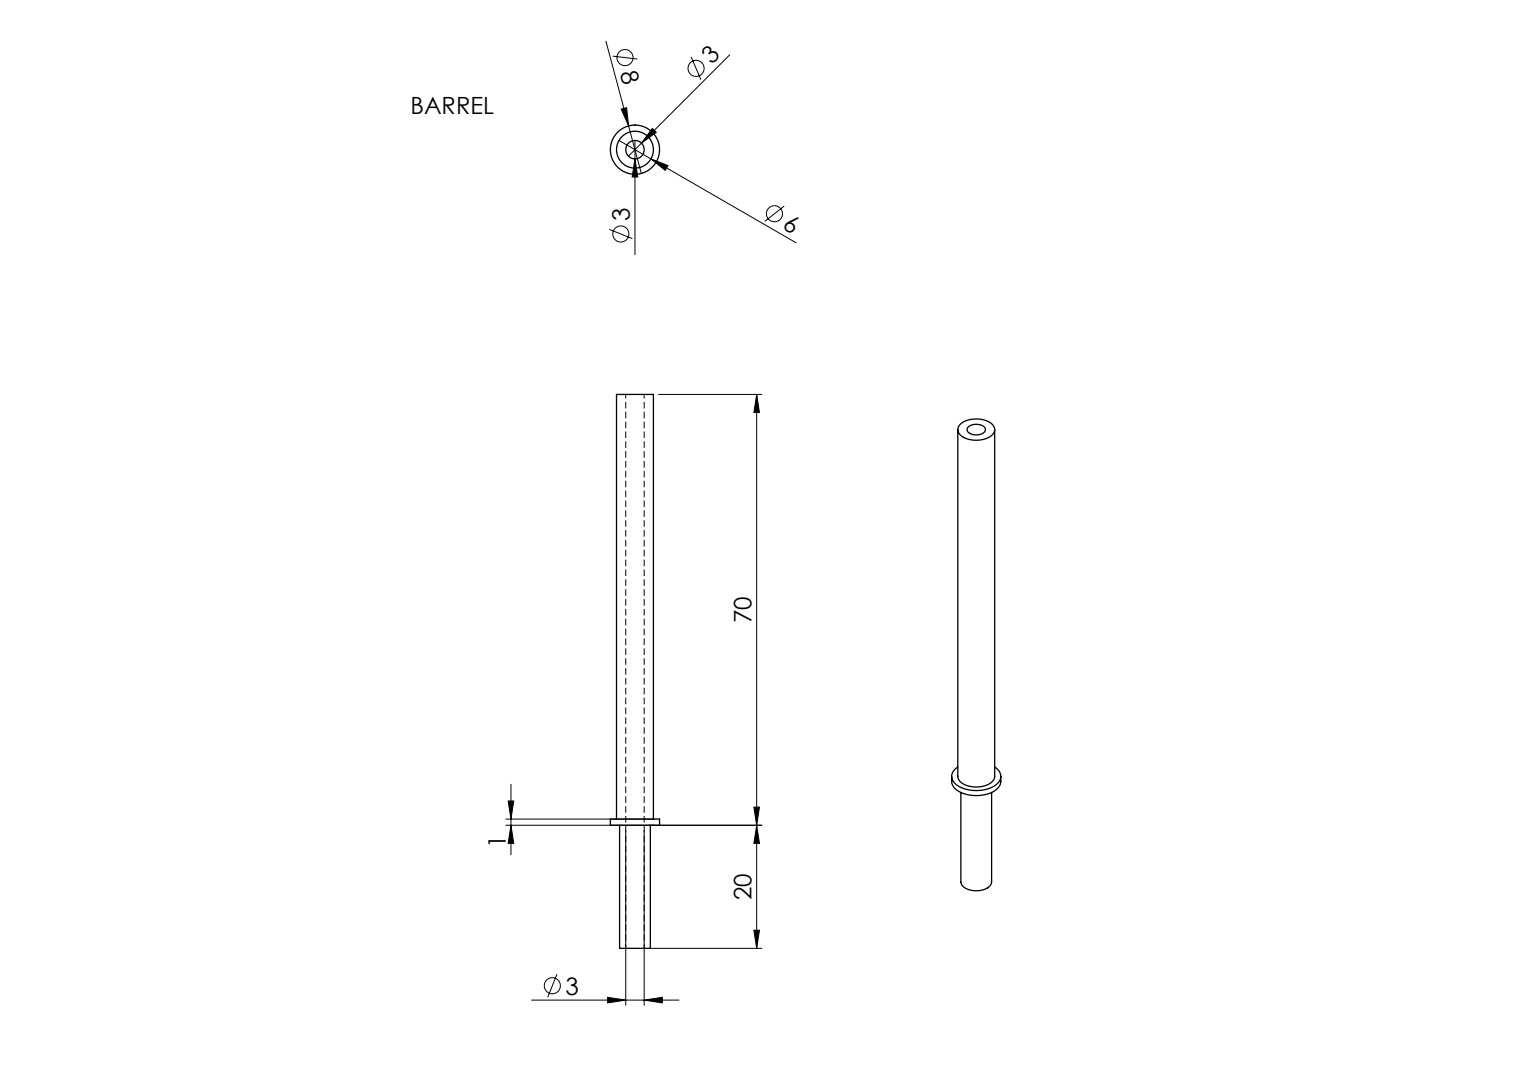
ISO-10303-21;
HEADER;
FILE_DESCRIPTION (('STEP AP214'),
    '1' );
FILE_NAME ('barrel.step',
    '2026-10-27T10:49:47',
    ( '' ),
    ( '' ),
    'SwSTEP 2.0',
    'SolidWorks 2026',
    '' );
FILE_SCHEMA (( 'AUTOMOTIVE_DESIGN' ));
ENDSEC;

DATA;
#22=EDGE_LOOP ( 'NONE', ( #1173, #7087 ) ) ;
#35=ADVANCED_FACE ( 'NONE', ( #4002 ), #1115, .T. ) ;
#54=CIRCLE ( 'NONE', #4368, 3.000000000000000444 ) ;
#95=( NAMED_UNIT ( * ) SI_UNIT ( $, .STERADIAN. ) SOLID_ANGLE_UNIT ( ) );
#116=VERTEX_POINT ( 'NONE', #4866 ) ;
#117=DIRECTION ( 'NONE',  ( 0.000000000000000000, -0.000000000000000000, 1.000000000000000000 ) ) ;
#151=DIRECTION ( 'NONE',  ( 0.000000000000000000, -1.000000000000000000, 0.000000000000000000 ) ) ;
#176=LINE ( 'NONE', #7340, #7480 ) ;
#209=DIRECTION ( 'NONE',  ( 0.000000000000000000, -1.000000000000000000, 0.000000000000000000 ) ) ;
#248=EDGE_CURVE ( 'NONE', #7024, #2834, #3444, .T. ) ;
#261=CARTESIAN_POINT ( 'NONE',  ( 0.000000000000000000, 1.000000000000000000, -3.999999999999999112 ) ) ;
#290=EDGE_CURVE ( 'NONE', #6114, #7024, #5977, .T. ) ;
#326=ORIENTED_EDGE ( 'NONE', *, *, #7017, .T. ) ;
#337=FACE_OUTER_BOUND ( 'NONE', #2501, .T. ) ;
#369=ORIENTED_EDGE ( 'NONE', *, *, #5900, .T. ) ;
#417=ADVANCED_BREP_SHAPE_REPRESENTATION ( '', ( #8468, #888 ), #7729 ) ;
#475=ORIENTED_EDGE ( 'NONE', *, *, #2084, .T. ) ;
#533=CARTESIAN_POINT ( 'NONE',  ( 0.000000000000000000, 70.00000000000000000, 0.000000000000000000 ) ) ;
#572=FACE_OUTER_BOUND ( 'NONE', #9117, .T. ) ;
#618=SURFACE_SIDE_STYLE ('',( #6992 ) ) ;
#623=( NAMED_UNIT ( * ) SI_UNIT ( $, .STERADIAN. ) SOLID_ANGLE_UNIT ( ) );
#637=DIRECTION ( 'NONE',  ( -0.000000000000000000, -1.000000000000000000, -0.000000000000000000 ) ) ;
#651=VECTOR ( 'NONE', #2655, 1000.000000000000000 ) ;
#686=DIRECTION ( 'NONE',  ( 0.000000000000000000, -1.000000000000000000, 0.000000000000000000 ) ) ;
#719=AXIS2_PLACEMENT_3D ( 'NONE', #7347, #8874, #4420 ) ;
#768=EDGE_CURVE ( 'NONE', #2834, #2260, #8516, .T. ) ;
#781=CARTESIAN_POINT ( 'NONE',  ( 3.061616997868383634E-16, -20.00000000000000000, -2.500000000000000444 ) ) ;
#835=ORIENTED_EDGE ( 'NONE', *, *, #8338, .F. ) ;
#878=CARTESIAN_POINT ( 'NONE',  ( 3.673940397442060361E-16, 70.00000000000000000, 3.000000000000000444 ) ) ;
#886=AXIS2_PLACEMENT_3D ( 'NONE', #6121, #3897, #6716 ) ;
#888=AXIS2_PLACEMENT_3D ( 'NONE', #4026, #9081, #6861 ) ;
#899=AXIS2_PLACEMENT_3D ( 'NONE', #5052, #7905, #6359 ) ;
#901=EDGE_CURVE ( 'NONE', #6843, #5960, #176, .T. ) ;
#910=CARTESIAN_POINT ( 'NONE',  ( 0.000000000000000000, 0.000000000000000000, 0.000000000000000000 ) ) ;
#921=CARTESIAN_POINT ( 'NONE',  ( 1.836970198721030181E-16, 70.00000000000000000, 1.500000000000000222 ) ) ;
#973=CARTESIAN_POINT ( 'NONE',  ( 4.898587196589411843E-16, 1.000000000000000000, 3.999999999999999112 ) ) ;
#1002=DIRECTION ( 'NONE',  ( 0.000000000000000000, -1.000000000000000000, 0.000000000000000000 ) ) ;
#1036=DIRECTION ( 'NONE',  ( 0.000000000000000000, 0.000000000000000000, -1.000000000000000000 ) ) ;
#1065=ORIENTED_EDGE ( 'NONE', *, *, #1265, .F. ) ;
#1115=CYLINDRICAL_SURFACE ( 'NONE', #2552, 3.999999999999999112 ) ;
#1139=ORIENTED_EDGE ( 'NONE', *, *, #8338, .T. ) ;
#1173=ORIENTED_EDGE ( 'NONE', *, *, #1265, .T. ) ;
#1220=ORIENTED_EDGE ( 'NONE', *, *, #6666, .T. ) ;
#1235=LINE ( 'NONE', #3240, #2069 ) ;
#1246=ORIENTED_EDGE ( 'NONE', *, *, #6279, .T. ) ;
#1265=EDGE_CURVE ( 'NONE', #2260, #2834, #6581, .T. ) ;
#1271=DIRECTION ( 'NONE',  ( -0.000000000000000000, -1.000000000000000000, -0.000000000000000000 ) ) ;
#1296=CARTESIAN_POINT ( 'NONE',  ( 3.673940397442060361E-16, 1.000000000000000888, 3.000000000000000444 ) ) ;
#1312=DIRECTION ( 'NONE',  ( -0.000000000000000000, -1.000000000000000000, -0.000000000000000000 ) ) ;
#1314=FILL_AREA_STYLE ('',( #8394 ) ) ;
#1334=CIRCLE ( 'NONE', #7748, 1.500000000000000222 ) ;
#1335=EDGE_CURVE ( 'NONE', #8226, #5826, #3482, .T. ) ;
#1339=PRODUCT_DEFINITION_CONTEXT ( 'detailed design', #4961, 'design' ) ;
#1343=AXIS2_PLACEMENT_3D ( 'NONE', #8806, #6806, #1036 ) ;
#1352=CYLINDRICAL_SURFACE ( 'NONE', #1343, 3.999999999999999112 ) ;
#1405=SURFACE_STYLE_USAGE ( .BOTH. , #618 ) ;
#1464=EDGE_CURVE ( 'NONE', #6101, #3013, #5044, .T. ) ;
#1479=CLOSED_SHELL ( 'NONE', ( #4412, #3247, #2822, #5525, #9073, #2667, #4256, #5038, #4493, #35, #5330, #3737 ) ) ;
#1506=EDGE_LOOP ( 'NONE', ( #5687, #3390 ) ) ;
#1527=DIRECTION ( 'NONE',  ( 0.000000000000000000, 1.000000000000000000, 0.000000000000000000 ) ) ;
#1576=ORIENTED_EDGE ( 'NONE', *, *, #1464, .F. ) ;
#1705=FACE_OUTER_BOUND ( 'NONE', #3131, .T. ) ;
#1741=ORIENTED_EDGE ( 'NONE', *, *, #768, .F. ) ;
#1746=CARTESIAN_POINT ( 'NONE',  ( 0.000000000000000000, 70.00000000000000000, 0.000000000000000000 ) ) ;
#1752=VERTEX_POINT ( 'NONE', #7681 ) ;
#1760=CARTESIAN_POINT ( 'NONE',  ( 0.000000000000000000, -20.00000000000000000, 0.000000000000000000 ) ) ;
#1766=CIRCLE ( 'NONE', #719, 2.500000000000000444 ) ;
#1768=ORIENTED_EDGE ( 'NONE', *, *, #2025, .T. ) ;
#1771=CARTESIAN_POINT ( 'NONE',  ( 1.836970198721030181E-16, -20.00000000000000000, 1.500000000000000222 ) ) ;
#1772=EDGE_LOOP ( 'NONE', ( #1220, #9002, #6481, #6040 ) ) ;
#1782=AXIS2_PLACEMENT_3D ( 'NONE', #3671, #1527, #4513 ) ;
#1783=EDGE_LOOP ( 'NONE', ( #3498, #8024, #3217, #7823 ) ) ;
#1815=DIRECTION ( 'NONE',  ( 0.000000000000000000, -1.000000000000000000, 0.000000000000000000 ) ) ;
#1830=EDGE_LOOP ( 'NONE', ( #3630, #6617, #3382, #8852 ) ) ;
#1889=DIRECTION ( 'NONE',  ( 0.000000000000000000, 0.000000000000000000, -1.000000000000000000 ) ) ;
#1906=AXIS2_PLACEMENT_3D ( 'NONE', #2039, #6307, #4863 ) ;
#1909=DIRECTION ( 'NONE',  ( -0.000000000000000000, 1.000000000000000000, -0.000000000000000000 ) ) ;
#1950=CARTESIAN_POINT ( 'NONE',  ( 3.061616997868383634E-16, -20.00000000000000000, -2.500000000000000444 ) ) ;
#1962=CARTESIAN_POINT ( 'NONE',  ( 1.836970198721030181E-16, 70.00000000000000000, 1.500000000000000222 ) ) ;
#1971=LINE ( 'NONE', #4800, #4797 ) ;
#1986=DIRECTION ( 'NONE',  ( 0.000000000000000000, 0.000000000000000000, -1.000000000000000000 ) ) ;
#1990=AXIS2_PLACEMENT_3D ( 'NONE', #8461, #2087, #4227 ) ;
#2025=EDGE_CURVE ( 'NONE', #7863, #6101, #7202, .T. ) ;
#2026=( NAMED_UNIT ( * ) PLANE_ANGLE_UNIT ( ) SI_UNIT ( $, .RADIAN. ) );
#2039=CARTESIAN_POINT ( 'NONE',  ( 0.000000000000000000, 0.000000000000000000, 0.000000000000000000 ) ) ;
#2065=DIRECTION ( 'NONE',  ( 0.000000000000000000, 1.000000000000000000, 0.000000000000000000 ) ) ;
#2069=VECTOR ( 'NONE', #7469, 1000.000000000000000 ) ;
#2083=VECTOR ( 'NONE', #6598, 1000.000000000000000 ) ;
#2084=EDGE_CURVE ( 'NONE', #5960, #5957, #3878, .T. ) ;
#2087=DIRECTION ( 'NONE',  ( 0.000000000000000000, -1.000000000000000000, 0.000000000000000000 ) ) ;
#2156=CYLINDRICAL_SURFACE ( 'NONE', #4658, 1.500000000000000222 ) ;
#2260=VERTEX_POINT ( 'NONE', #8456 ) ;
#2273=DIRECTION ( 'NONE',  ( -0.000000000000000000, -1.000000000000000000, -0.000000000000000000 ) ) ;
#2276=ORIENTED_EDGE ( 'NONE', *, *, #7313, .F. ) ;
#2297=EDGE_CURVE ( 'NONE', #7186, #8226, #1334, .T. ) ;
#2310=DIRECTION ( 'NONE',  ( 0.000000000000000000, 1.000000000000000000, 0.000000000000000000 ) ) ;
#2334=CARTESIAN_POINT ( 'NONE',  ( 0.000000000000000000, -20.00000000000000000, -1.500000000000000222 ) ) ;
#2347=ORIENTED_EDGE ( 'NONE', *, *, #2994, .T. ) ;
#2360=CIRCLE ( 'NONE', #3409, 1.500000000000000222 ) ;
#2381=AXIS2_PLACEMENT_3D ( 'NONE', #8404, #6381, #1986 ) ;
#2460=DIRECTION ( 'NONE',  ( 1.000000000000000000, 0.000000000000000000, 0.000000000000000000 ) ) ;
#2501=EDGE_LOOP ( 'NONE', ( #7351, #2982, #1065, #4344 ) ) ;
#2541=DIRECTION ( 'NONE',  ( 0.000000000000000000, 0.000000000000000000, 1.000000000000000000 ) ) ;
#2552=AXIS2_PLACEMENT_3D ( 'NONE', #6080, #1815, #3168 ) ;
#2585=FACE_BOUND ( 'NONE', #4396, .T. ) ;
#2612=CARTESIAN_POINT ( 'NONE',  ( 0.000000000000000000, -20.00000000000000000, 0.000000000000000000 ) ) ;
#2616=SHAPE_DEFINITION_REPRESENTATION ( #4672, #3200 ) ;
#2655=DIRECTION ( 'NONE',  ( 0.000000000000000000, -1.000000000000000000, 0.000000000000000000 ) ) ;
#2667=ADVANCED_FACE ( 'NONE', ( #1705, #6583 ), #7375, .T. ) ;
#2697=VECTOR ( 'NONE', #4369, 1000.000000000000000 ) ;
#2741=AXIS2_PLACEMENT_3D ( 'NONE', #6157, #3930, #4669 ) ;
#2788=CARTESIAN_POINT ( 'NONE',  ( 0.000000000000000000, 70.00000000000000000, 0.000000000000000000 ) ) ;
#2822=ADVANCED_FACE ( 'NONE', ( #3293 ), #4681, .F. ) ;
#2834=VERTEX_POINT ( 'NONE', #5371 ) ;
#2864=FACE_OUTER_BOUND ( 'NONE', #22, .T. ) ;
#2928=CARTESIAN_POINT ( 'NONE',  ( 3.061616997868383634E-16, 0.000000000000000000, -2.500000000000000444 ) ) ;
#2945=PRODUCT_DEFINITION_FORMATION_WITH_SPECIFIED_SOURCE ( 'ANY', '', #8393, .NOT_KNOWN. ) ;
#2948=MECHANICAL_DESIGN_GEOMETRIC_PRESENTATION_REPRESENTATION('',(#5632),#3563);
#2959=ORIENTED_EDGE ( 'NONE', *, *, #7430, .T. ) ;
#2960=ORIENTED_EDGE ( 'NONE', *, *, #6666, .F. ) ;
#2982=ORIENTED_EDGE ( 'NONE', *, *, #248, .T. ) ;
#2994=EDGE_CURVE ( 'NONE', #7024, #6114, #3567, .T. ) ;
#3001=DIRECTION ( 'NONE',  ( 0.000000000000000000, -0.000000000000000000, -1.000000000000000000 ) ) ;
#3013=VERTEX_POINT ( 'NONE', #4897 ) ;
#3051=DIRECTION ( 'NONE',  ( -0.000000000000000000, 1.000000000000000000, -0.000000000000000000 ) ) ;
#3092=FACE_OUTER_BOUND ( 'NONE', #1506, .T. ) ;
#3095=CARTESIAN_POINT ( 'NONE',  ( 0.000000000000000000, 1.000000000000000888, 0.000000000000000000 ) ) ;
#3131=EDGE_LOOP ( 'NONE', ( #8535, #369 ) ) ;
#3168=DIRECTION ( 'NONE',  ( 0.000000000000000000, 0.000000000000000000, -1.000000000000000000 ) ) ;
#3180=CIRCLE ( 'NONE', #4212, 3.000000000000000444 ) ;
#3191=DIRECTION ( 'NONE',  ( 0.000000000000000000, -1.000000000000000000, 0.000000000000000000 ) ) ;
#3200=SHAPE_REPRESENTATION ( 'barrel', ( #888 ), #7729 ) ;
#3217=ORIENTED_EDGE ( 'NONE', *, *, #5142, .F. ) ;
#3240=CARTESIAN_POINT ( 'NONE',  ( 0.000000000000000000, -20.00000000000000000, 2.500000000000000444 ) ) ;
#3247=ADVANCED_FACE ( 'NONE', ( #337 ), #1352, .T. ) ;
#3258=CARTESIAN_POINT ( 'NONE',  ( 0.000000000000000000, 70.00000000000000000, 0.000000000000000000 ) ) ;
#3263=ORIENTED_EDGE ( 'NONE', *, *, #248, .F. ) ;
#3274=AXIS2_PLACEMENT_3D ( 'NONE', #5839, #2310, #117 ) ;
#3278=EDGE_CURVE ( 'NONE', #5826, #6937, #5346, .T. ) ;
#3279=COLOUR_RGB ( '',0.8941176470588234615, 0.8941176470588234615, 0.8941176470588234615 ) ;
#3293=FACE_OUTER_BOUND ( 'NONE', #1772, .T. ) ;
#3302=FACE_OUTER_BOUND ( 'NONE', #6606, .T. ) ;
#3382=ORIENTED_EDGE ( 'NONE', *, *, #4776, .T. ) ;
#3390=ORIENTED_EDGE ( 'NONE', *, *, #2994, .F. ) ;
#3409=AXIS2_PLACEMENT_3D ( 'NONE', #1746, #6762, #2541 ) ;
#3420=( NAMED_UNIT ( * ) PLANE_ANGLE_UNIT ( ) SI_UNIT ( $, .RADIAN. ) );
#3444=LINE ( 'NONE', #5613, #8804 ) ;
#3460=DIRECTION ( 'NONE',  ( 0.000000000000000000, 0.000000000000000000, -1.000000000000000000 ) ) ;
#3466=PLANE ( 'NONE',  #3609 ) ;
#3482=LINE ( 'NONE', #3615, #4273 ) ;
#3486=PRODUCT_DEFINITION ( 'UNKNOWN', '', #2945, #1339 ) ;
#3498=ORIENTED_EDGE ( 'NONE', *, *, #5900, .F. ) ;
#3510=( LENGTH_UNIT ( ) NAMED_UNIT ( * ) SI_UNIT ( .MILLI., .METRE. ) );
#3547=CIRCLE ( 'NONE', #7110, 1.500000000000000222 ) ;
#3563=( GEOMETRIC_REPRESENTATION_CONTEXT ( 3 ) GLOBAL_UNCERTAINTY_ASSIGNED_CONTEXT ( ( #7291 ) ) GLOBAL_UNIT_ASSIGNED_CONTEXT ( ( #3510, #2026, #623 ) ) REPRESENTATION_CONTEXT ( 'NONE', 'WORKASPACE' ) );
#3567=CIRCLE ( 'NONE', #2381, 3.999999999999999112 ) ;
#3609=AXIS2_PLACEMENT_3D ( 'NONE', #9087, #2065, #5021 ) ;
#3615=CARTESIAN_POINT ( 'NONE',  ( 0.000000000000000000, 70.00000000000000000, -1.500000000000000222 ) ) ;
#3630=ORIENTED_EDGE ( 'NONE', *, *, #901, .F. ) ;
#3671=CARTESIAN_POINT ( 'NONE',  ( 0.000000000000000000, 70.00000000000000000, 0.000000000000000000 ) ) ;
#3675=MECHANICAL_DESIGN_GEOMETRIC_PRESENTATION_REPRESENTATION('',(#9162),#7384);
#3737=ADVANCED_FACE ( 'NONE', ( #3302 ), #8963, .T. ) ;
#3751=DIRECTION ( 'NONE',  ( 1.000000000000000000, 0.000000000000000000, 0.000000000000000000 ) ) ;
#3775=AXIS2_PLACEMENT_3D ( 'NONE', #8021, #209, #3751 ) ;
#3806=EDGE_LOOP ( 'NONE', ( #2960, #7095 ) ) ;
#3878=CIRCLE ( 'NONE', #899, 3.000000000000000444 ) ;
#3897=DIRECTION ( 'NONE',  ( -0.000000000000000000, -1.000000000000000000, -0.000000000000000000 ) ) ;
#3930=DIRECTION ( 'NONE',  ( 0.000000000000000000, -1.000000000000000000, 0.000000000000000000 ) ) ;
#3931=CIRCLE ( 'NONE', #3775, 2.500000000000000444 ) ;
#3989=ORIENTED_EDGE ( 'NONE', *, *, #9010, .F. ) ;
#4001=LINE ( 'NONE', #8138, #651 ) ;
#4002=FACE_OUTER_BOUND ( 'NONE', #4221, .T. ) ;
#4026=CARTESIAN_POINT ( 'NONE',  ( 0.000000000000000000, 0.000000000000000000, 0.000000000000000000 ) ) ;
#4056=ORIENTED_EDGE ( 'NONE', *, *, #2297, .T. ) ;
#4157=CYLINDRICAL_SURFACE ( 'NONE', #6087, 3.000000000000000444 ) ;
#4164=FACE_OUTER_BOUND ( 'NONE', #5923, .T. ) ;
#4198=CARTESIAN_POINT ( 'NONE',  ( 0.000000000000000000, 70.00000000000000000, 0.000000000000000000 ) ) ;
#4212=AXIS2_PLACEMENT_3D ( 'NONE', #3095, #8665, #6010 ) ;
#4221=EDGE_LOOP ( 'NONE', ( #3263, #2347, #5735, #1741 ) ) ;
#4227=DIRECTION ( 'NONE',  ( 0.000000000000000000, 0.000000000000000000, -1.000000000000000000 ) ) ;
#4256=ADVANCED_FACE ( 'NONE', ( #6376, #2864 ), #3466, .F. ) ;
#4273=VECTOR ( 'NONE', #637, 1000.000000000000000 ) ;
#4318=CARTESIAN_POINT ( 'NONE',  ( 0.000000000000000000, -20.00000000000000000, 0.000000000000000000 ) ) ;
#4334=CYLINDRICAL_SURFACE ( 'NONE', #4517, 3.000000000000000444 ) ;
#4344=ORIENTED_EDGE ( 'NONE', *, *, #5766, .F. ) ;
#4368=AXIS2_PLACEMENT_3D ( 'NONE', #3258, #6083, #8919 ) ;
#4369=DIRECTION ( 'NONE',  ( -0.000000000000000000, 1.000000000000000000, -0.000000000000000000 ) ) ;
#4382=PRESENTATION_STYLE_ASSIGNMENT (( #1405 ) ) ;
#4396=EDGE_LOOP ( 'NONE', ( #6921, #2276 ) ) ;
#4412=ADVANCED_FACE ( 'NONE', ( #4164 ), #6998, .T. ) ;
#4420=DIRECTION ( 'NONE',  ( 1.000000000000000000, 0.000000000000000000, 0.000000000000000000 ) ) ;
#4493=ADVANCED_FACE ( 'NONE', ( #3092, #7176 ), #5772, .F. ) ;
#4513=DIRECTION ( 'NONE',  ( 0.000000000000000000, 0.000000000000000000, 1.000000000000000000 ) ) ;
#4517=AXIS2_PLACEMENT_3D ( 'NONE', #4198, #1312, #7166 ) ;
#4658=AXIS2_PLACEMENT_3D ( 'NONE', #8527, #4934, #6293 ) ;
#4669=DIRECTION ( 'NONE',  ( 0.000000000000000000, -0.000000000000000000, -1.000000000000000000 ) ) ;
#4672=PRODUCT_DEFINITION_SHAPE ( 'NONE', 'NONE',  #3486 ) ;
#4681=CYLINDRICAL_SURFACE ( 'NONE', #886, 1.500000000000000222 ) ;
#4700=ORIENTED_EDGE ( 'NONE', *, *, #2025, .F. ) ;
#4734=DIRECTION ( 'NONE',  ( 0.000000000000000000, 0.000000000000000000, 1.000000000000000000 ) ) ;
#4776=EDGE_CURVE ( 'NONE', #1752, #5957, #1971, .T. ) ;
#4785=PRODUCT_CONTEXT ( 'NONE', #5448, 'mechanical' ) ;
#4797=VECTOR ( 'NONE', #1271, 1000.000000000000000 ) ;
#4800=CARTESIAN_POINT ( 'NONE',  ( 0.000000000000000000, 70.00000000000000000, -3.000000000000000444 ) ) ;
#4863=DIRECTION ( 'NONE',  ( 0.000000000000000000, 0.000000000000000000, -1.000000000000000000 ) ) ;
#4866=CARTESIAN_POINT ( 'NONE',  ( 0.000000000000000000, -20.00000000000000000, 2.500000000000000444 ) ) ;
#4878=CARTESIAN_POINT ( 'NONE',  ( 0.000000000000000000, -20.00000000000000000, 0.000000000000000000 ) ) ;
#4897=CARTESIAN_POINT ( 'NONE',  ( 0.000000000000000000, 0.000000000000000000, 2.500000000000000444 ) ) ;
#4934=DIRECTION ( 'NONE',  ( -0.000000000000000000, -1.000000000000000000, -0.000000000000000000 ) ) ;
#4961=APPLICATION_CONTEXT ( 'automotive_design' ) ;
#5021=DIRECTION ( 'NONE',  ( 0.000000000000000000, -0.000000000000000000, 1.000000000000000000 ) ) ;
#5038=ADVANCED_FACE ( 'NONE', ( #7040 ), #2156, .F. ) ;
#5044=CIRCLE ( 'NONE', #8916, 2.500000000000000444 ) ;
#5052=CARTESIAN_POINT ( 'NONE',  ( 0.000000000000000000, 1.000000000000000888, 0.000000000000000000 ) ) ;
#5060=ORIENTED_EDGE ( 'NONE', *, *, #6279, .F. ) ;
#5084=AXIS2_PLACEMENT_3D ( 'NONE', #5639, #3051, #5868 ) ;
#5142=EDGE_CURVE ( 'NONE', #5957, #5960, #3180, .T. ) ;
#5287=DIRECTION ( 'NONE',  ( 0.000000000000000000, 0.000000000000000000, -1.000000000000000000 ) ) ;
#5330=ADVANCED_FACE ( 'NONE', ( #572, #2585 ), #9031, .T. ) ;
#5346=CIRCLE ( 'NONE', #6093, 1.500000000000000222 ) ;
#5371=CARTESIAN_POINT ( 'NONE',  ( 4.898587196589411843E-16, 0.000000000000000000, 3.999999999999999112 ) ) ;
#5448=APPLICATION_CONTEXT ( 'automotive_design' ) ;
#5507=FACE_OUTER_BOUND ( 'NONE', #1830, .T. ) ;
#5525=ADVANCED_FACE ( 'NONE', ( #8562 ), #4334, .T. ) ;
#5530=DIRECTION ( 'NONE',  ( 0.000000000000000000, -1.000000000000000000, 0.000000000000000000 ) ) ;
#5613=CARTESIAN_POINT ( 'NONE',  ( 4.898587196589411843E-16, 1.000000000000000000, 3.999999999999999112 ) ) ;
#5632=STYLED_ITEM('',(#9218),#8468);
#5633=SHAPE_REPRESENTATION_RELATIONSHIP ( 'NONE' , 'NONE' ,  #3200, #417 ) ;
#5639=CARTESIAN_POINT ( 'NONE',  ( 0.000000000000000000, -20.00000000000000000, 0.000000000000000000 ) ) ;
#5687=ORIENTED_EDGE ( 'NONE', *, *, #290, .F. ) ;
#5735=ORIENTED_EDGE ( 'NONE', *, *, #5766, .T. ) ;
#5766=EDGE_CURVE ( 'NONE', #6114, #2260, #4001, .T. ) ;
#5772=PLANE ( 'NONE',  #6282 ) ;
#5818=( LENGTH_UNIT ( ) NAMED_UNIT ( * ) SI_UNIT ( .MILLI., .METRE. ) );
#5826=VERTEX_POINT ( 'NONE', #2334 ) ;
#5837=CARTESIAN_POINT ( 'NONE',  ( 0.000000000000000000, 70.00000000000000000, -1.500000000000000222 ) ) ;
#5839=CARTESIAN_POINT ( 'NONE',  ( 0.000000000000000000, 70.00000000000000000, 0.000000000000000000 ) ) ;
#5868=DIRECTION ( 'NONE',  ( 0.000000000000000000, 0.000000000000000000, 1.000000000000000000 ) ) ;
#5891=UNCERTAINTY_MEASURE_WITH_UNIT (LENGTH_MEASURE( 1.000000000000000082E-05 ), #6946, 'distance_accuracy_value', 'NONE');
#5900=EDGE_CURVE ( 'NONE', #6843, #1752, #54, .T. ) ;
#5923=EDGE_LOOP ( 'NONE', ( #9154, #1768, #7664, #835 ) ) ;
#5957=VERTEX_POINT ( 'NONE', #7060 ) ;
#5960=VERTEX_POINT ( 'NONE', #1296 ) ;
#5975=DIRECTION ( 'NONE',  ( 1.000000000000000000, 0.000000000000000000, 0.000000000000000000 ) ) ;
#5977=CIRCLE ( 'NONE', #1990, 3.999999999999999112 ) ;
#6010=DIRECTION ( 'NONE',  ( 0.000000000000000000, 0.000000000000000000, -1.000000000000000000 ) ) ;
#6040=ORIENTED_EDGE ( 'NONE', *, *, #1335, .F. ) ;
#6080=CARTESIAN_POINT ( 'NONE',  ( 0.000000000000000000, 1.000000000000000000, 0.000000000000000000 ) ) ;
#6083=DIRECTION ( 'NONE',  ( 0.000000000000000000, 1.000000000000000000, 0.000000000000000000 ) ) ;
#6087=AXIS2_PLACEMENT_3D ( 'NONE', #533, #6161, #3460 ) ;
#6093=AXIS2_PLACEMENT_3D ( 'NONE', #4878, #3191, #1889 ) ;
#6101=VERTEX_POINT ( 'NONE', #2928 ) ;
#6114=VERTEX_POINT ( 'NONE', #261 ) ;
#6121=CARTESIAN_POINT ( 'NONE',  ( 0.000000000000000000, 70.00000000000000000, 0.000000000000000000 ) ) ;
#6157=CARTESIAN_POINT ( 'NONE',  ( 0.000000000000000000, -20.00000000000000000, 0.000000000000000000 ) ) ;
#6161=DIRECTION ( 'NONE',  ( -0.000000000000000000, -1.000000000000000000, -0.000000000000000000 ) ) ;
#6279=EDGE_CURVE ( 'NONE', #116, #7863, #3931, .T. ) ;
#6282=AXIS2_PLACEMENT_3D ( 'NONE', #6514, #151, #3001 ) ;
#6293=DIRECTION ( 'NONE',  ( 0.000000000000000000, 0.000000000000000000, -1.000000000000000000 ) ) ;
#6307=DIRECTION ( 'NONE',  ( 0.000000000000000000, -1.000000000000000000, 0.000000000000000000 ) ) ;
#6314=DIRECTION ( 'NONE',  ( 0.000000000000000000, 0.000000000000000000, -1.000000000000000000 ) ) ;
#6359=DIRECTION ( 'NONE',  ( 0.000000000000000000, 0.000000000000000000, -1.000000000000000000 ) ) ;
#6376=FACE_BOUND ( 'NONE', #7465, .T. ) ;
#6381=DIRECTION ( 'NONE',  ( 0.000000000000000000, -1.000000000000000000, 0.000000000000000000 ) ) ;
#6436=ORIENTED_EDGE ( 'NONE', *, *, #1335, .T. ) ;
#6481=ORIENTED_EDGE ( 'NONE', *, *, #7313, .T. ) ;
#6514=CARTESIAN_POINT ( 'NONE',  ( 0.000000000000000000, 1.000000000000000000, 0.000000000000000000 ) ) ;
#6539=UNCERTAINTY_MEASURE_WITH_UNIT (LENGTH_MEASURE( 1.000000000000000082E-05 ), #5818, 'distance_accuracy_value', 'NONE');
#6581=CIRCLE ( 'NONE', #1906, 3.999999999999999112 ) ;
#6583=FACE_BOUND ( 'NONE', #3806, .T. ) ;
#6598=DIRECTION ( 'NONE',  ( -0.000000000000000000, -1.000000000000000000, -0.000000000000000000 ) ) ;
#6606=EDGE_LOOP ( 'NONE', ( #4700, #5060, #1139, #326 ) ) ;
#6617=ORIENTED_EDGE ( 'NONE', *, *, #8913, .F. ) ;
#6637=DIRECTION ( 'NONE',  ( 0.000000000000000000, -1.000000000000000000, 0.000000000000000000 ) ) ;
#6663=AXIS2_PLACEMENT_3D ( 'NONE', #1760, #7434, #2460 ) ;
#6664=EDGE_LOOP ( 'NONE', ( #8316, #475 ) ) ;
#6666=EDGE_CURVE ( 'NONE', #8226, #7186, #2360, .T. ) ;
#6716=DIRECTION ( 'NONE',  ( 0.000000000000000000, 0.000000000000000000, -1.000000000000000000 ) ) ;
#6762=DIRECTION ( 'NONE',  ( 0.000000000000000000, 1.000000000000000000, 0.000000000000000000 ) ) ;
#6806=DIRECTION ( 'NONE',  ( 0.000000000000000000, -1.000000000000000000, 0.000000000000000000 ) ) ;
#6843=VERTEX_POINT ( 'NONE', #878 ) ;
#6861=DIRECTION ( 'NONE',  ( 1.000000000000000000, 0.000000000000000000, 0.000000000000000000 ) ) ;
#6901=ORIENTED_EDGE ( 'NONE', *, *, #7017, .F. ) ;
#6921=ORIENTED_EDGE ( 'NONE', *, *, #3278, .F. ) ;
#6937=VERTEX_POINT ( 'NONE', #1771 ) ;
#6946=( LENGTH_UNIT ( ) NAMED_UNIT ( * ) SI_UNIT ( .MILLI., .METRE. ) );
#6992=SURFACE_STYLE_FILL_AREA ( #1314 ) ;
#6998=CYLINDRICAL_SURFACE ( 'NONE', #5084, 2.500000000000000444 ) ;
#7017=EDGE_CURVE ( 'NONE', #3013, #6101, #1766, .T. ) ;
#7024=VERTEX_POINT ( 'NONE', #973 ) ;
#7040=FACE_OUTER_BOUND ( 'NONE', #8700, .T. ) ;
#7054=DIRECTION ( 'NONE',  ( 0.000000000000000000, 1.000000000000000000, 0.000000000000000000 ) ) ;
#7060=CARTESIAN_POINT ( 'NONE',  ( 0.000000000000000000, 1.000000000000000888, -3.000000000000000444 ) ) ;
#7087=ORIENTED_EDGE ( 'NONE', *, *, #768, .T. ) ;
#7095=ORIENTED_EDGE ( 'NONE', *, *, #2297, .F. ) ;
#7110=AXIS2_PLACEMENT_3D ( 'NONE', #4318, #686, #6314 ) ;
#7166=DIRECTION ( 'NONE',  ( 0.000000000000000000, 0.000000000000000000, -1.000000000000000000 ) ) ;
#7170=( NAMED_UNIT ( * ) PLANE_ANGLE_UNIT ( ) SI_UNIT ( $, .RADIAN. ) );
#7175=AXIS2_PLACEMENT_3D ( 'NONE', #8039, #6637, #5287 ) ;
#7176=FACE_BOUND ( 'NONE', #6664, .T. ) ;
#7186=VERTEX_POINT ( 'NONE', #1962 ) ;
#7202=LINE ( 'NONE', #781, #2697 ) ;
#7291=UNCERTAINTY_MEASURE_WITH_UNIT (LENGTH_MEASURE( 1.000000000000000082E-05 ), #3510, 'distance_accuracy_value', 'NONE');
#7297=LINE ( 'NONE', #921, #2083 ) ;
#7313=EDGE_CURVE ( 'NONE', #6937, #5826, #3547, .T. ) ;
#7340=CARTESIAN_POINT ( 'NONE',  ( 3.673940397442060361E-16, 70.00000000000000000, 3.000000000000000444 ) ) ;
#7347=CARTESIAN_POINT ( 'NONE',  ( 0.000000000000000000, 0.000000000000000000, 0.000000000000000000 ) ) ;
#7351=ORIENTED_EDGE ( 'NONE', *, *, #290, .T. ) ;
#7375=PLANE ( 'NONE',  #3274 ) ;
#7384=( GEOMETRIC_REPRESENTATION_CONTEXT ( 3 ) GLOBAL_UNCERTAINTY_ASSIGNED_CONTEXT ( ( #6539 ) ) GLOBAL_UNIT_ASSIGNED_CONTEXT ( ( #5818, #7170, #95 ) ) REPRESENTATION_CONTEXT ( 'NONE', 'WORKASPACE' ) );
#7430=EDGE_CURVE ( 'NONE', #7863, #116, #8004, .T. ) ;
#7434=DIRECTION ( 'NONE',  ( 0.000000000000000000, -1.000000000000000000, 0.000000000000000000 ) ) ;
#7465=EDGE_LOOP ( 'NONE', ( #6901, #1576 ) ) ;
#7469=DIRECTION ( 'NONE',  ( -0.000000000000000000, 1.000000000000000000, -0.000000000000000000 ) ) ;
#7480=VECTOR ( 'NONE', #2273, 1000.000000000000000 ) ;
#7556=( NAMED_UNIT ( * ) SI_UNIT ( $, .STERADIAN. ) SOLID_ANGLE_UNIT ( ) );
#7664=ORIENTED_EDGE ( 'NONE', *, *, #1464, .T. ) ;
#7681=CARTESIAN_POINT ( 'NONE',  ( 0.000000000000000000, 70.00000000000000000, -3.000000000000000444 ) ) ;
#7729=( GEOMETRIC_REPRESENTATION_CONTEXT ( 3 ) GLOBAL_UNCERTAINTY_ASSIGNED_CONTEXT ( ( #5891 ) ) GLOBAL_UNIT_ASSIGNED_CONTEXT ( ( #6946, #3420, #7556 ) ) REPRESENTATION_CONTEXT ( 'NONE', 'WORKASPACE' ) );
#7748=AXIS2_PLACEMENT_3D ( 'NONE', #2788, #7054, #8502 ) ;
#7823=ORIENTED_EDGE ( 'NONE', *, *, #4776, .F. ) ;
#7863=VERTEX_POINT ( 'NONE', #1950 ) ;
#7905=DIRECTION ( 'NONE',  ( 0.000000000000000000, -1.000000000000000000, 0.000000000000000000 ) ) ;
#8004=CIRCLE ( 'NONE', #6663, 2.500000000000000444 ) ;
#8021=CARTESIAN_POINT ( 'NONE',  ( 0.000000000000000000, -20.00000000000000000, 0.000000000000000000 ) ) ;
#8024=ORIENTED_EDGE ( 'NONE', *, *, #901, .T. ) ;
#8039=CARTESIAN_POINT ( 'NONE',  ( 0.000000000000000000, 0.000000000000000000, 0.000000000000000000 ) ) ;
#8138=CARTESIAN_POINT ( 'NONE',  ( 0.000000000000000000, 1.000000000000000000, -3.999999999999999112 ) ) ;
#8226=VERTEX_POINT ( 'NONE', #5837 ) ;
#8316=ORIENTED_EDGE ( 'NONE', *, *, #5142, .T. ) ;
#8327=AXIS2_PLACEMENT_3D ( 'NONE', #2612, #1909, #4734 ) ;
#8338=EDGE_CURVE ( 'NONE', #116, #3013, #1235, .T. ) ;
#8393=PRODUCT ( 'barrel', 'barrel', '', ( #4785 ) ) ;
#8394=FILL_AREA_STYLE_COLOUR ( '', #3279 ) ;
#8404=CARTESIAN_POINT ( 'NONE',  ( 0.000000000000000000, 1.000000000000000000, 0.000000000000000000 ) ) ;
#8456=CARTESIAN_POINT ( 'NONE',  ( 0.000000000000000000, 0.000000000000000000, -3.999999999999999112 ) ) ;
#8461=CARTESIAN_POINT ( 'NONE',  ( 0.000000000000000000, 1.000000000000000000, 0.000000000000000000 ) ) ;
#8468=MANIFOLD_SOLID_BREP ( 'Extrude-Thin1', #1479 ) ;
#8502=DIRECTION ( 'NONE',  ( 0.000000000000000000, 0.000000000000000000, 1.000000000000000000 ) ) ;
#8516=CIRCLE ( 'NONE', #7175, 3.999999999999999112 ) ;
#8527=CARTESIAN_POINT ( 'NONE',  ( 0.000000000000000000, 70.00000000000000000, 0.000000000000000000 ) ) ;
#8535=ORIENTED_EDGE ( 'NONE', *, *, #8913, .T. ) ;
#8562=FACE_OUTER_BOUND ( 'NONE', #1783, .T. ) ;
#8609=CIRCLE ( 'NONE', #1782, 3.000000000000000444 ) ;
#8665=DIRECTION ( 'NONE',  ( 0.000000000000000000, -1.000000000000000000, 0.000000000000000000 ) ) ;
#8697=ORIENTED_EDGE ( 'NONE', *, *, #3278, .T. ) ;
#8700=EDGE_LOOP ( 'NONE', ( #3989, #4056, #6436, #8697 ) ) ;
#8804=VECTOR ( 'NONE', #5530, 1000.000000000000000 ) ;
#8806=CARTESIAN_POINT ( 'NONE',  ( 0.000000000000000000, 1.000000000000000000, 0.000000000000000000 ) ) ;
#8852=ORIENTED_EDGE ( 'NONE', *, *, #2084, .F. ) ;
#8874=DIRECTION ( 'NONE',  ( 0.000000000000000000, -1.000000000000000000, 0.000000000000000000 ) ) ;
#8913=EDGE_CURVE ( 'NONE', #1752, #6843, #8609, .T. ) ;
#8916=AXIS2_PLACEMENT_3D ( 'NONE', #910, #1002, #5975 ) ;
#8919=DIRECTION ( 'NONE',  ( 0.000000000000000000, 0.000000000000000000, 1.000000000000000000 ) ) ;
#8963=CYLINDRICAL_SURFACE ( 'NONE', #8327, 2.500000000000000444 ) ;
#9002=ORIENTED_EDGE ( 'NONE', *, *, #9010, .T. ) ;
#9010=EDGE_CURVE ( 'NONE', #7186, #6937, #7297, .T. ) ;
#9031=PLANE ( 'NONE',  #2741 ) ;
#9073=ADVANCED_FACE ( 'NONE', ( #5507 ), #4157, .T. ) ;
#9081=DIRECTION ( 'NONE',  ( 0.000000000000000000, 0.000000000000000000, 1.000000000000000000 ) ) ;
#9087=CARTESIAN_POINT ( 'NONE',  ( 0.000000000000000000, 0.000000000000000000, 0.000000000000000000 ) ) ;
#9117=EDGE_LOOP ( 'NONE', ( #1246, #2959 ) ) ;
#9154=ORIENTED_EDGE ( 'NONE', *, *, #7430, .F. ) ;
#9162=STYLED_ITEM ( 'NONE', ( #4382 ), #417 ) ;
#9212=COLOUR_RGB('Sky Blue',0.24,0.69,0.87);
#9213=FILL_AREA_STYLE_COLOUR('',#9212);
#9214=FILL_AREA_STYLE('',(#9213));
#9215=SURFACE_STYLE_FILL_AREA(#9214);
#9216=SURFACE_SIDE_STYLE('',(#9215));
#9217=SURFACE_STYLE_USAGE(.BOTH.,#9216);
#9218=PRESENTATION_STYLE_ASSIGNMENT((#9217));
ENDSEC;
END-ISO-10303-21;
